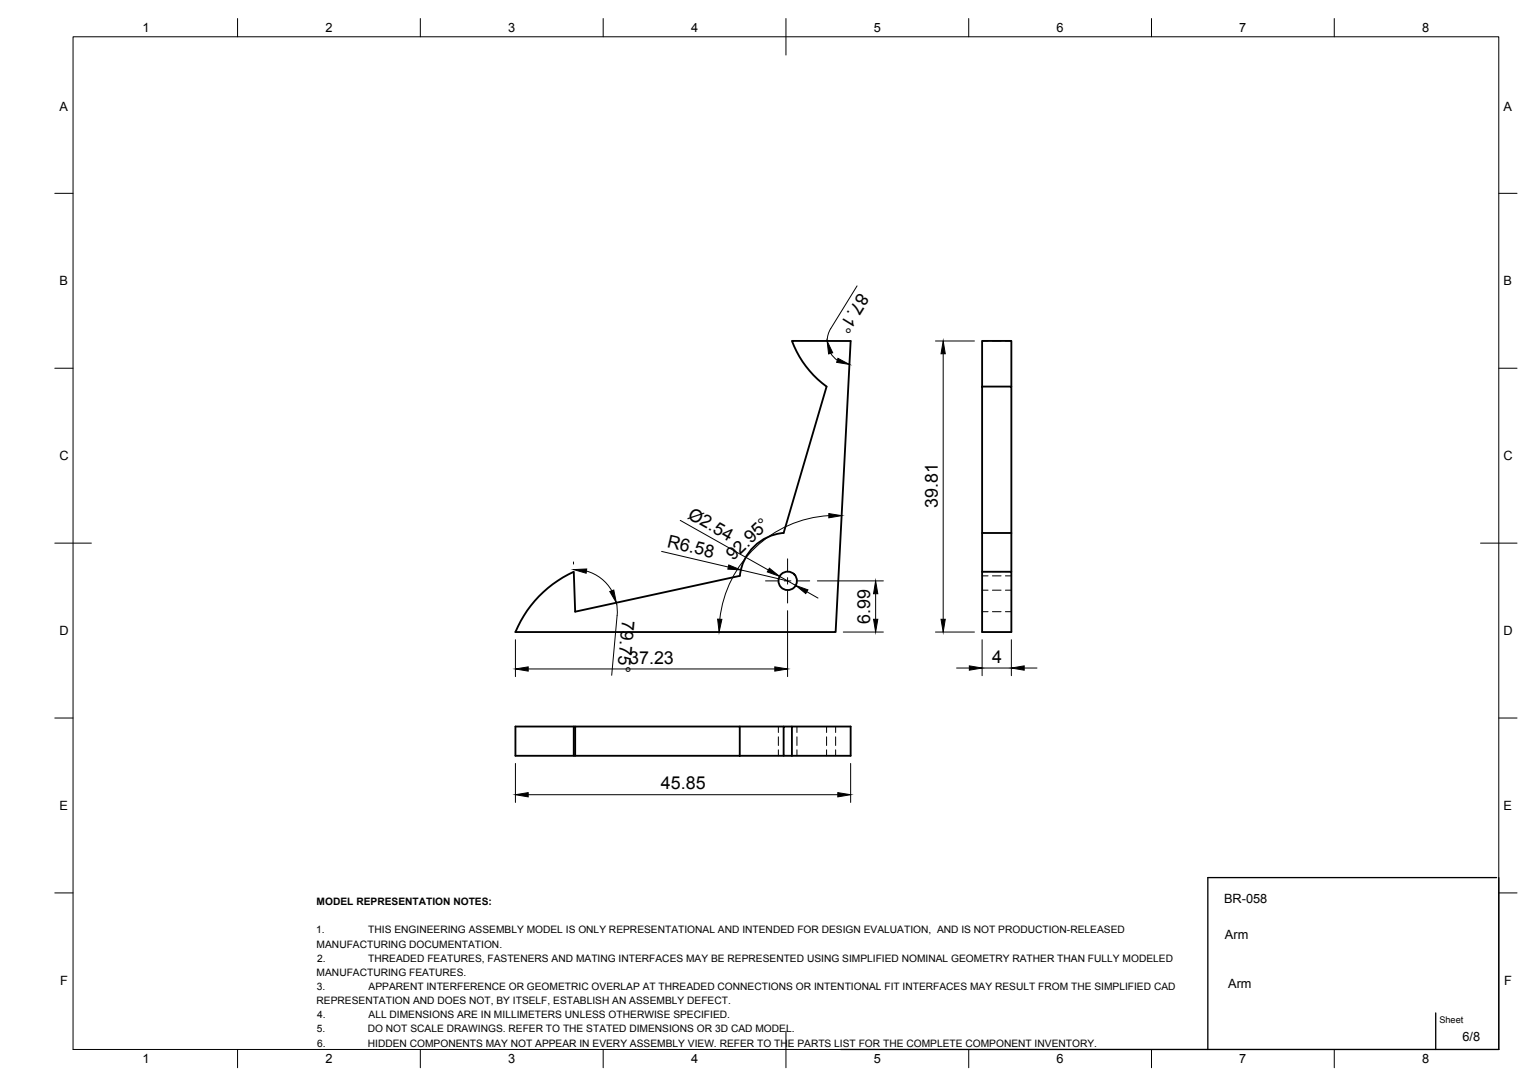
ISO-10303-21;
HEADER;
/* Generated by software containing ST-Developer
 * from STEP Tools, Inc. (www.steptools.com) 
 */

FILE_DESCRIPTION(
/* description */ (''),
/* implementation_level */ '2;1');

FILE_NAME(
/* name */ 'Arm.step',
/* time_stamp */ '2026-10-12T16:07:47-07:00',
/* author */ (''),
/* organization */ (''),
/* preprocessor_version */ 'ST-DEVELOPER v20.2',
/* originating_system */ 'Autodesk Translation Framework v15.15.0.0',
/* authorisation */ '');

FILE_SCHEMA (('AUTOMOTIVE_DESIGN { 1 0 10303 214 3 1 1 }'));
ENDSEC;

DATA;
#10=MECHANICAL_DESIGN_GEOMETRIC_PRESENTATION_REPRESENTATION('',(#96),#8779);
#82=SHAPE_REPRESENTATION_RELATIONSHIP('SRR','None',#8811,#89);
#89=ADVANCED_BREP_SHAPE_REPRESENTATION('',(#106),#8774);
#96=STYLED_ITEM('',(#8855),#106);
#106=MANIFOLD_SOLID_BREP('Body1',#5116);
#148=FACE_BOUND('',#987,.T.);
#149=FACE_BOUND('',#989,.T.);
#293=CIRCLE('',#5523,6.58030196793658);
#294=CIRCLE('',#5524,6.58030196793658);
#295=CIRCLE('',#5528,1.26938918348039);
#296=CIRCLE('',#5529,1.26938918348039);
#297=CIRCLE('',#5532,13.6540067108022);
#298=CIRCLE('',#5533,13.6540067108022);
#299=CIRCLE('',#5536,15.694333954976);
#300=CIRCLE('',#5537,15.694333954976);
#458=CYLINDRICAL_SURFACE('',#5522,6.58030196793658);
#459=CYLINDRICAL_SURFACE('',#5527,1.26938918348039);
#460=CYLINDRICAL_SURFACE('',#5531,13.6540067108022);
#461=CYLINDRICAL_SURFACE('',#5535,15.694333954976);
#665=FACE_OUTER_BOUND('',#976,.T.);
#666=FACE_OUTER_BOUND('',#977,.T.);
#667=FACE_OUTER_BOUND('',#978,.T.);
#668=FACE_OUTER_BOUND('',#979,.T.);
#669=FACE_OUTER_BOUND('',#980,.T.);
#670=FACE_OUTER_BOUND('',#981,.T.);
#671=FACE_OUTER_BOUND('',#982,.T.);
#672=FACE_OUTER_BOUND('',#983,.T.);
#673=FACE_OUTER_BOUND('',#984,.T.);
#674=FACE_OUTER_BOUND('',#985,.T.);
#675=FACE_OUTER_BOUND('',#986,.T.);
#676=FACE_OUTER_BOUND('',#988,.T.);
#976=EDGE_LOOP('',(#4356,#4357,#4358,#4359));
#977=EDGE_LOOP('',(#4360,#4361,#4362,#4363));
#978=EDGE_LOOP('',(#4364,#4365,#4366,#4367));
#979=EDGE_LOOP('',(#4368,#4369,#4370,#4371));
#980=EDGE_LOOP('',(#4372,#4373,#4374,#4375));
#981=EDGE_LOOP('',(#4376,#4377,#4378,#4379));
#982=EDGE_LOOP('',(#4380,#4381,#4382,#4383));
#983=EDGE_LOOP('',(#4384,#4385,#4386,#4387));
#984=EDGE_LOOP('',(#4388,#4389,#4390,#4391));
#985=EDGE_LOOP('',(#4392,#4393,#4394,#4395));
#986=EDGE_LOOP('',(#4396,#4397,#4398,#4399,#4400,#4401,#4402,#4403,#4404));
#987=EDGE_LOOP('',(#4405));
#988=EDGE_LOOP('',(#4406,#4407,#4408,#4409,#4410,#4411,#4412,#4413,#4414));
#989=EDGE_LOOP('',(#4415));
#1518=LINE('',#8374,#2003);
#1519=LINE('',#8376,#2004);
#1520=LINE('',#8378,#2005);
#1521=LINE('',#8379,#2006);
#1522=LINE('',#8383,#2007);
#1523=LINE('',#8385,#2008);
#1524=LINE('',#8387,#2009);
#1525=LINE('',#8388,#2010);
#1526=LINE('',#8395,#2011);
#1527=LINE('',#8397,#2012);
#1528=LINE('',#8399,#2013);
#1529=LINE('',#8400,#2014);
#1530=LINE('',#8403,#2015);
#1531=LINE('',#8405,#2016);
#1532=LINE('',#8406,#2017);
#1533=LINE('',#8411,#2018);
#1534=LINE('',#8415,#2019);
#1535=LINE('',#8417,#2020);
#1536=LINE('',#8418,#2021);
#1537=LINE('',#8424,#2022);
#1538=LINE('',#8426,#2023);
#1539=LINE('',#8427,#2024);
#2003=VECTOR('',#6794,10.);
#2004=VECTOR('',#6795,10.);
#2005=VECTOR('',#6796,10.);
#2006=VECTOR('',#6797,10.);
#2007=VECTOR('',#6800,10.);
#2008=VECTOR('',#6801,10.);
#2009=VECTOR('',#6802,10.);
#2010=VECTOR('',#6803,10.);
#2011=VECTOR('',#6812,10.);
#2012=VECTOR('',#6813,10.);
#2013=VECTOR('',#6814,10.);
#2014=VECTOR('',#6815,10.);
#2015=VECTOR('',#6818,10.);
#2016=VECTOR('',#6819,10.);
#2017=VECTOR('',#6820,10.);
#2018=VECTOR('',#6825,1.26938918348039);
#2019=VECTOR('',#6830,10.);
#2020=VECTOR('',#6831,10.);
#2021=VECTOR('',#6832,10.);
#2022=VECTOR('',#6841,10.);
#2023=VECTOR('',#6842,10.);
#2024=VECTOR('',#6843,10.);
#2426=VERTEX_POINT('',#8372);
#2427=VERTEX_POINT('',#8373);
#2428=VERTEX_POINT('',#8375);
#2429=VERTEX_POINT('',#8377);
#2430=VERTEX_POINT('',#8381);
#2431=VERTEX_POINT('',#8382);
#2432=VERTEX_POINT('',#8384);
#2433=VERTEX_POINT('',#8386);
#2434=VERTEX_POINT('',#8393);
#2435=VERTEX_POINT('',#8394);
#2436=VERTEX_POINT('',#8396);
#2437=VERTEX_POINT('',#8398);
#2438=VERTEX_POINT('',#8402);
#2439=VERTEX_POINT('',#8404);
#2440=VERTEX_POINT('',#8408);
#2441=VERTEX_POINT('',#8410);
#2442=VERTEX_POINT('',#8414);
#2443=VERTEX_POINT('',#8416);
#2444=VERTEX_POINT('',#8423);
#2445=VERTEX_POINT('',#8425);
#3082=EDGE_CURVE('',#2426,#2427,#1518,.T.);
#3083=EDGE_CURVE('',#2426,#2428,#1519,.T.);
#3084=EDGE_CURVE('',#2429,#2428,#1520,.T.);
#3085=EDGE_CURVE('',#2429,#2427,#1521,.T.);
#3086=EDGE_CURVE('',#2430,#2431,#1522,.T.);
#3087=EDGE_CURVE('',#2432,#2431,#1523,.T.);
#3088=EDGE_CURVE('',#2433,#2432,#1524,.T.);
#3089=EDGE_CURVE('',#2430,#2433,#1525,.T.);
#3090=EDGE_CURVE('',#2430,#2426,#293,.T.);
#3091=EDGE_CURVE('',#2428,#2433,#294,.T.);
#3092=EDGE_CURVE('',#2434,#2435,#1526,.T.);
#3093=EDGE_CURVE('',#2436,#2435,#1527,.T.);
#3094=EDGE_CURVE('',#2437,#2436,#1528,.T.);
#3095=EDGE_CURVE('',#2434,#2437,#1529,.T.);
#3096=EDGE_CURVE('',#2434,#2438,#1530,.T.);
#3097=EDGE_CURVE('',#2439,#2437,#1531,.T.);
#3098=EDGE_CURVE('',#2439,#2438,#1532,.T.);
#3099=EDGE_CURVE('',#2440,#2440,#295,.T.);
#3100=EDGE_CURVE('',#2440,#2441,#1533,.T.);
#3101=EDGE_CURVE('',#2441,#2441,#296,.T.);
#3102=EDGE_CURVE('',#2436,#2442,#1534,.T.);
#3103=EDGE_CURVE('',#2443,#2435,#1535,.T.);
#3104=EDGE_CURVE('',#2442,#2443,#1536,.T.);
#3105=EDGE_CURVE('',#2442,#2429,#297,.T.);
#3106=EDGE_CURVE('',#2427,#2443,#298,.T.);
#3107=EDGE_CURVE('',#2444,#2432,#1537,.F.);
#3108=EDGE_CURVE('',#2445,#2431,#1538,.T.);
#3109=EDGE_CURVE('',#2444,#2445,#1539,.T.);
#3110=EDGE_CURVE('',#2444,#2439,#299,.T.);
#3111=EDGE_CURVE('',#2438,#2445,#300,.T.);
#4356=ORIENTED_EDGE('',*,*,#3082,.F.);
#4357=ORIENTED_EDGE('',*,*,#3083,.T.);
#4358=ORIENTED_EDGE('',*,*,#3084,.F.);
#4359=ORIENTED_EDGE('',*,*,#3085,.T.);
#4360=ORIENTED_EDGE('',*,*,#3086,.T.);
#4361=ORIENTED_EDGE('',*,*,#3087,.F.);
#4362=ORIENTED_EDGE('',*,*,#3088,.F.);
#4363=ORIENTED_EDGE('',*,*,#3089,.F.);
#4364=ORIENTED_EDGE('',*,*,#3090,.F.);
#4365=ORIENTED_EDGE('',*,*,#3089,.T.);
#4366=ORIENTED_EDGE('',*,*,#3091,.F.);
#4367=ORIENTED_EDGE('',*,*,#3083,.F.);
#4368=ORIENTED_EDGE('',*,*,#3092,.T.);
#4369=ORIENTED_EDGE('',*,*,#3093,.F.);
#4370=ORIENTED_EDGE('',*,*,#3094,.F.);
#4371=ORIENTED_EDGE('',*,*,#3095,.F.);
#4372=ORIENTED_EDGE('',*,*,#3096,.F.);
#4373=ORIENTED_EDGE('',*,*,#3095,.T.);
#4374=ORIENTED_EDGE('',*,*,#3097,.F.);
#4375=ORIENTED_EDGE('',*,*,#3098,.T.);
#4376=ORIENTED_EDGE('',*,*,#3099,.F.);
#4377=ORIENTED_EDGE('',*,*,#3100,.T.);
#4378=ORIENTED_EDGE('',*,*,#3101,.F.);
#4379=ORIENTED_EDGE('',*,*,#3100,.F.);
#4380=ORIENTED_EDGE('',*,*,#3102,.F.);
#4381=ORIENTED_EDGE('',*,*,#3093,.T.);
#4382=ORIENTED_EDGE('',*,*,#3103,.F.);
#4383=ORIENTED_EDGE('',*,*,#3104,.F.);
#4384=ORIENTED_EDGE('',*,*,#3105,.F.);
#4385=ORIENTED_EDGE('',*,*,#3104,.T.);
#4386=ORIENTED_EDGE('',*,*,#3106,.F.);
#4387=ORIENTED_EDGE('',*,*,#3085,.F.);
#4388=ORIENTED_EDGE('',*,*,#3107,.T.);
#4389=ORIENTED_EDGE('',*,*,#3087,.T.);
#4390=ORIENTED_EDGE('',*,*,#3108,.F.);
#4391=ORIENTED_EDGE('',*,*,#3109,.F.);
#4392=ORIENTED_EDGE('',*,*,#3110,.F.);
#4393=ORIENTED_EDGE('',*,*,#3109,.T.);
#4394=ORIENTED_EDGE('',*,*,#3111,.F.);
#4395=ORIENTED_EDGE('',*,*,#3098,.F.);
#4396=ORIENTED_EDGE('',*,*,#3102,.T.);
#4397=ORIENTED_EDGE('',*,*,#3105,.T.);
#4398=ORIENTED_EDGE('',*,*,#3084,.T.);
#4399=ORIENTED_EDGE('',*,*,#3091,.T.);
#4400=ORIENTED_EDGE('',*,*,#3088,.T.);
#4401=ORIENTED_EDGE('',*,*,#3107,.F.);
#4402=ORIENTED_EDGE('',*,*,#3110,.T.);
#4403=ORIENTED_EDGE('',*,*,#3097,.T.);
#4404=ORIENTED_EDGE('',*,*,#3094,.T.);
#4405=ORIENTED_EDGE('',*,*,#3099,.T.);
#4406=ORIENTED_EDGE('',*,*,#3111,.T.);
#4407=ORIENTED_EDGE('',*,*,#3108,.T.);
#4408=ORIENTED_EDGE('',*,*,#3086,.F.);
#4409=ORIENTED_EDGE('',*,*,#3090,.T.);
#4410=ORIENTED_EDGE('',*,*,#3082,.T.);
#4411=ORIENTED_EDGE('',*,*,#3106,.T.);
#4412=ORIENTED_EDGE('',*,*,#3103,.T.);
#4413=ORIENTED_EDGE('',*,*,#3092,.F.);
#4414=ORIENTED_EDGE('',*,*,#3096,.T.);
#4415=ORIENTED_EDGE('',*,*,#3101,.T.);
#4800=PLANE('',#5520);
#4801=PLANE('',#5521);
#4802=PLANE('',#5525);
#4803=PLANE('',#5526);
#4804=PLANE('',#5530);
#4805=PLANE('',#5534);
#4806=PLANE('',#5538);
#4807=PLANE('',#5539);
#5027=ADVANCED_FACE('',(#665),#4800,.T.);
#5028=ADVANCED_FACE('',(#666),#4801,.T.);
#5029=ADVANCED_FACE('',(#667),#458,.T.);
#5030=ADVANCED_FACE('',(#668),#4802,.T.);
#5031=ADVANCED_FACE('',(#669),#4803,.T.);
#5032=ADVANCED_FACE('',(#670),#459,.F.);
#5033=ADVANCED_FACE('',(#671),#4804,.T.);
#5034=ADVANCED_FACE('',(#672),#460,.T.);
#5035=ADVANCED_FACE('',(#673),#4805,.T.);
#5036=ADVANCED_FACE('',(#674),#461,.T.);
#5037=ADVANCED_FACE('',(#675,#148),#4806,.T.);
#5038=ADVANCED_FACE('',(#676,#149),#4807,.F.);
#5116=CLOSED_SHELL('',(#5027,#5028,#5029,#5030,#5031,#5032,#5033,#5034,
#5035,#5036,#5037,#5038));
#5519=AXIS2_PLACEMENT_3D('',#8370,#6790,#6791);
#5520=AXIS2_PLACEMENT_3D('',#8371,#6792,#6793);
#5521=AXIS2_PLACEMENT_3D('',#8380,#6798,#6799);
#5522=AXIS2_PLACEMENT_3D('',#8389,#6804,#6805);
#5523=AXIS2_PLACEMENT_3D('',#8390,#6806,#6807);
#5524=AXIS2_PLACEMENT_3D('',#8391,#6808,#6809);
#5525=AXIS2_PLACEMENT_3D('',#8392,#6810,#6811);
#5526=AXIS2_PLACEMENT_3D('',#8401,#6816,#6817);
#5527=AXIS2_PLACEMENT_3D('',#8407,#6821,#6822);
#5528=AXIS2_PLACEMENT_3D('',#8409,#6823,#6824);
#5529=AXIS2_PLACEMENT_3D('',#8412,#6826,#6827);
#5530=AXIS2_PLACEMENT_3D('',#8413,#6828,#6829);
#5531=AXIS2_PLACEMENT_3D('',#8419,#6833,#6834);
#5532=AXIS2_PLACEMENT_3D('',#8420,#6835,#6836);
#5533=AXIS2_PLACEMENT_3D('',#8421,#6837,#6838);
#5534=AXIS2_PLACEMENT_3D('',#8422,#6839,#6840);
#5535=AXIS2_PLACEMENT_3D('',#8428,#6844,#6845);
#5536=AXIS2_PLACEMENT_3D('',#8429,#6846,#6847);
#5537=AXIS2_PLACEMENT_3D('',#8430,#6848,#6849);
#5538=AXIS2_PLACEMENT_3D('',#8431,#6850,#6851);
#5539=AXIS2_PLACEMENT_3D('',#8432,#6852,#6853);
#6790=DIRECTION('axis',(0.,0.,1.));
#6791=DIRECTION('refdir',(1.,0.,0.));
#6792=DIRECTION('center_axis',(-0.506446725163971,0.,-0.862271253475778));
#6793=DIRECTION('ref_axis',(-0.862271253475778,0.,0.506446725163971));
#6794=DIRECTION('',(0.862271253475778,0.,-0.506446725163971));
#6795=DIRECTION('',(0.,1.,0.));
#6796=DIRECTION('',(-0.862271253475778,0.,0.506446725163971));
#6797=DIRECTION('',(0.,-1.,0.));
#6798=DIRECTION('center_axis',(0.514130343945888,0.,-0.857712066741563));
#6799=DIRECTION('ref_axis',(-0.857712066741563,0.,-0.514130343945888));
#6800=DIRECTION('',(-0.857712066741563,0.,-0.514130343945888));
#6801=DIRECTION('',(0.,-1.,0.));
#6802=DIRECTION('',(-0.857712066741563,0.,-0.514130343945888));
#6803=DIRECTION('',(0.,1.,0.));
#6804=DIRECTION('center_axis',(0.,1.,0.));
#6805=DIRECTION('ref_axis',(-0.65291015697706,0.,-0.757435361543274));
#6806=DIRECTION('center_axis',(0.,-1.,0.));
#6807=DIRECTION('ref_axis',(-0.65291015697706,0.,-0.757435361543274));
#6808=DIRECTION('center_axis',(0.,1.,0.));
#6809=DIRECTION('ref_axis',(-0.65291015697706,0.,-0.757435361543274));
#6810=DIRECTION('center_axis',(0.692652702068206,0.,0.72127126264507));
#6811=DIRECTION('ref_axis',(0.72127126264507,0.,-0.692652702068206));
#6812=DIRECTION('',(0.72127126264507,0.,-0.692652702068206));
#6813=DIRECTION('',(0.,-1.,0.));
#6814=DIRECTION('',(0.72127126264507,0.,-0.692652702068206));
#6815=DIRECTION('',(0.,1.,0.));
#6816=DIRECTION('center_axis',(-0.684689477581543,0.,0.728834905372345));
#6817=DIRECTION('ref_axis',(0.728834905372345,0.,0.684689477581543));
#6818=DIRECTION('',(-0.728834905372345,0.,-0.684689477581542));
#6819=DIRECTION('',(0.728834905372345,0.,0.684689477581542));
#6820=DIRECTION('',(0.,-1.,0.));
#6821=DIRECTION('center_axis',(0.,-1.,0.));
#6822=DIRECTION('ref_axis',(1.,0.,0.));
#6823=DIRECTION('center_axis',(0.,-1.,0.));
#6824=DIRECTION('ref_axis',(1.,0.,0.));
#6825=DIRECTION('',(0.,-1.,0.));
#6826=DIRECTION('center_axis',(0.,1.,0.));
#6827=DIRECTION('ref_axis',(1.,0.,0.));
#6828=DIRECTION('center_axis',(0.685364699004991,0.,-0.728199992692803));
#6829=DIRECTION('ref_axis',(0.728199992692803,0.,0.685364699004991));
#6830=DIRECTION('',(-0.728199992692803,0.,-0.685364699004991));
#6831=DIRECTION('',(0.728199992692803,0.,0.685364699004991));
#6832=DIRECTION('',(0.,-1.,0.));
#6833=DIRECTION('center_axis',(0.,-1.,0.));
#6834=DIRECTION('ref_axis',(-0.922431509667951,0.,-0.38616073074784));
#6835=DIRECTION('center_axis',(0.,1.,0.));
#6836=DIRECTION('ref_axis',(-0.922431509667951,0.,-0.38616073074784));
#6837=DIRECTION('center_axis',(0.,-1.,0.));
#6838=DIRECTION('ref_axis',(-0.922431509667951,0.,-0.38616073074784));
#6839=DIRECTION('center_axis',(0.752564828001213,0.,0.658518169571277));
#6840=DIRECTION('ref_axis',(-0.658518169571277,0.,0.752564828001213));
#6841=DIRECTION('',(0.658518169571277,0.,-0.752564828001213));
#6842=DIRECTION('',(-0.658518169571277,0.,0.752564828001213));
#6843=DIRECTION('',(0.,-1.,0.));
#6844=DIRECTION('center_axis',(0.,-1.,0.));
#6845=DIRECTION('ref_axis',(0.321121156101037,0.,-0.947038121251903));
#6846=DIRECTION('center_axis',(0.,1.,0.));
#6847=DIRECTION('ref_axis',(0.321121156101037,0.,-0.947038121251903));
#6848=DIRECTION('center_axis',(0.,-1.,0.));
#6849=DIRECTION('ref_axis',(0.321121156101037,0.,-0.947038121251903));
#6850=DIRECTION('center_axis',(0.,1.,0.));
#6851=DIRECTION('ref_axis',(1.,0.,0.));
#6852=DIRECTION('center_axis',(0.,1.,0.));
#6853=DIRECTION('ref_axis',(1.,0.,0.));
#8370=CARTESIAN_POINT('',(0.,0.,0.));
#8371=CARTESIAN_POINT('Origin',(22.0759476067182,-6.5,76.7431289545307));
#8372=CARTESIAN_POINT('',(4.09006724262322,-6.5,87.3069627514587));
#8373=CARTESIAN_POINT('',(22.0759476067182,-6.5,76.7431289545307));
#8374=CARTESIAN_POINT('',(4.09006724262322,-6.5,87.3069627514587));
#8375=CARTESIAN_POINT('',(4.09006724262321,-2.5,87.3069627514587));
#8376=CARTESIAN_POINT('',(4.09006724262322,-6.5,87.3069627514587));
#8377=CARTESIAN_POINT('',(22.0759476067182,-2.5,76.7431289545307));
#8378=CARTESIAN_POINT('',(11.5910700858341,-2.5,82.9013208956311));
#8379=CARTESIAN_POINT('',(22.0759476067182,-4.5,76.7431289545307));
#8380=CARTESIAN_POINT('Origin',(-4.29634599084193,-6.5,87.477586159287));
#8381=CARTESIAN_POINT('',(-4.29634599084193,-6.5,87.477586159287));
#8382=CARTESIAN_POINT('',(-24.0531806351797,-6.5,75.634931048273));
#8383=CARTESIAN_POINT('',(-4.29634599084193,-6.5,87.477586159287));
#8384=CARTESIAN_POINT('',(-24.0531806351797,-2.5,75.634931048273));
#8385=CARTESIAN_POINT('',(-24.0531806351797,-4.5,75.634931048273));
#8386=CARTESIAN_POINT('',(-4.29634599084193,-2.5,87.477586159287));
#8387=CARTESIAN_POINT('',(-3.96187942842657,-2.5,87.6780723310932));
#8388=CARTESIAN_POINT('',(-4.29634599084193,-6.5,87.477586159287));
#8389=CARTESIAN_POINT('Origin',(0.,-6.5,92.461739559435));
#8390=CARTESIAN_POINT('Origin',(0.,-6.5,92.461739559435));
#8391=CARTESIAN_POINT('Origin',(0.,-2.5,92.461739559435));
#8392=CARTESIAN_POINT('Origin',(0.,-6.5,102.055558916393));
#8393=CARTESIAN_POINT('',(0.,-6.5,102.055558916393));
#8394=CARTESIAN_POINT('',(28.7457294952528,-6.5,74.4504008586727));
#8395=CARTESIAN_POINT('',(0.,-6.5,102.055558916393));
#8396=CARTESIAN_POINT('',(28.7457294952528,-2.5,74.4504008586727));
#8397=CARTESIAN_POINT('',(28.7457294952528,-4.5,74.4504008586727));
#8398=CARTESIAN_POINT('',(0.,-2.5,102.055558916393));
#8399=CARTESIAN_POINT('',(3.97893495048528,-2.5,98.234499922998));
#8400=CARTESIAN_POINT('',(0.,-6.5,102.055558916393));
#8401=CARTESIAN_POINT('Origin',(-31.9194481137532,-6.5,72.0694672890556));
#8402=CARTESIAN_POINT('',(-31.9194481137532,-6.5,72.0694672890556));
#8403=CARTESIAN_POINT('',(0.,-6.5,102.055558916393));
#8404=CARTESIAN_POINT('',(-31.9194481137532,-2.5,72.0694672890556));
#8405=CARTESIAN_POINT('',(-20.7679309766169,-2.5,82.545538600386));
#8406=CARTESIAN_POINT('',(-31.9194481137532,-4.5,72.0694672890556));
#8407=CARTESIAN_POINT('Origin',(0.,-4.5,92.461739559435));
#8408=CARTESIAN_POINT('',(-1.26938918348039,-2.5,92.461739559435));
#8409=CARTESIAN_POINT('Origin',(0.,-2.5,92.461739559435));
#8410=CARTESIAN_POINT('',(-1.26938918348039,-6.5,92.461739559435));
#8411=CARTESIAN_POINT('',(-1.26938918348039,-4.5,92.461739559435));
#8412=CARTESIAN_POINT('Origin',(0.,-6.5,92.461739559435));
#8413=CARTESIAN_POINT('Origin',(22.9001701836232,-4.5,68.948697977139));
#8414=CARTESIAN_POINT('',(22.9001701836232,-2.5,68.948697977139));
#8415=CARTESIAN_POINT('',(20.2820284879064,-2.5,66.4845646164644));
#8416=CARTESIAN_POINT('',(22.9001701836232,-6.5,68.948697977139));
#8417=CARTESIAN_POINT('',(28.7457294952528,-6.5,74.4504008586727));
#8418=CARTESIAN_POINT('',(22.9001701836232,-4.5,68.948697977139));
#8419=CARTESIAN_POINT('Origin',(35.4950562068848,-4.5,74.2213391862183));
#8420=CARTESIAN_POINT('Origin',(35.4950562068848,-2.5,74.2213391862183));
#8421=CARTESIAN_POINT('Origin',(35.4950562068848,-6.5,74.2213391862183));
#8422=CARTESIAN_POINT('Origin',(-20.4586462226688,-4.5,71.5270410964181));
#8423=CARTESIAN_POINT('',(-20.4586462226688,-2.5,71.5270410964181));
#8424=CARTESIAN_POINT('',(-19.5750050436382,-2.5,70.5172021843879));
#8425=CARTESIAN_POINT('',(-20.4586462226688,-6.5,71.5270410964181));
#8426=CARTESIAN_POINT('',(-20.4586462226688,-6.5,71.5270410964181));
#8427=CARTESIAN_POINT('',(-20.4586462226688,-4.5,71.5270410964181));
#8428=CARTESIAN_POINT('Origin',(-25.4984288865264,-4.5,86.3901736394385));
#8429=CARTESIAN_POINT('Origin',(-25.4984288865264,-2.5,86.3901736394385));
#8430=CARTESIAN_POINT('Origin',(-25.4984288865264,-6.5,86.3901736394385));
#8431=CARTESIAN_POINT('Origin',(-1.5868593092502,-2.5,84.4743489885695));
#8432=CARTESIAN_POINT('Origin',(-1.5868593092502,-6.5,84.4743489885695));
#8765=UNCERTAINTY_MEASURE_WITH_UNIT(LENGTH_MEASURE(0.01),#8780,
'DISTANCE_ACCURACY_VALUE',
'Maximum model space distance between geometric entities at asserted c
onnectivities');
#8770=UNCERTAINTY_MEASURE_WITH_UNIT(LENGTH_MEASURE(0.01),#8780,
'DISTANCE_ACCURACY_VALUE',
'Maximum model space distance between geometric entities at asserted c
onnectivities');
#8774=(
GEOMETRIC_REPRESENTATION_CONTEXT(3)
GLOBAL_UNCERTAINTY_ASSIGNED_CONTEXT((#8765))
GLOBAL_UNIT_ASSIGNED_CONTEXT((#8780,#8782,#8783))
REPRESENTATION_CONTEXT('','3D')
);
#8779=(
GEOMETRIC_REPRESENTATION_CONTEXT(3)
GLOBAL_UNCERTAINTY_ASSIGNED_CONTEXT((#8770))
GLOBAL_UNIT_ASSIGNED_CONTEXT((#8780,#8782,#8783))
REPRESENTATION_CONTEXT('','3D')
);
#8780=(
LENGTH_UNIT()
NAMED_UNIT(*)
SI_UNIT(.MILLI.,.METRE.)
);
#8782=(
NAMED_UNIT(*)
PLANE_ANGLE_UNIT()
SI_UNIT($,.RADIAN.)
);
#8783=(
NAMED_UNIT(*)
SI_UNIT($,.STERADIAN.)
SOLID_ANGLE_UNIT()
);
#8787=SHAPE_DEFINITION_REPRESENTATION(#8795,#8811);
#8795=PRODUCT_DEFINITION_SHAPE('',$,#8820);
#8811=SHAPE_REPRESENTATION('',(#5519),#8774);
#8816=PRODUCT_DEFINITION_CONTEXT('part definition',#8842,'design');
#8820=PRODUCT_DEFINITION('Arm','Arm',#8828,#8816);
#8828=PRODUCT_DEFINITION_FORMATION('',$,#8847);
#8842=APPLICATION_CONTEXT(
'Core Data for Automotive Mechanical Design Process');
#8843=PRODUCT_CONTEXT('part definition',#8842,'mechanical');
#8847=PRODUCT('Arm','Arm',$,(#8843));
#8855=PRESENTATION_STYLE_ASSIGNMENT((#8860));
#8860=SURFACE_STYLE_USAGE(.BOTH.,#8865);
#8865=SURFACE_SIDE_STYLE('',(#8870));
#8870=SURFACE_STYLE_FILL_AREA(#8875);
#8875=FILL_AREA_STYLE('Opaque(85,255,0)',(#8880));
#8880=FILL_AREA_STYLE_COLOUR('Opaque(85,255,0)',#8885);
#8885=COLOUR_RGB('Opaque(85,255,0)', 0.31764706, 0.68627451, 0.89019608);
ENDSEC;
END-ISO-10303-21;
